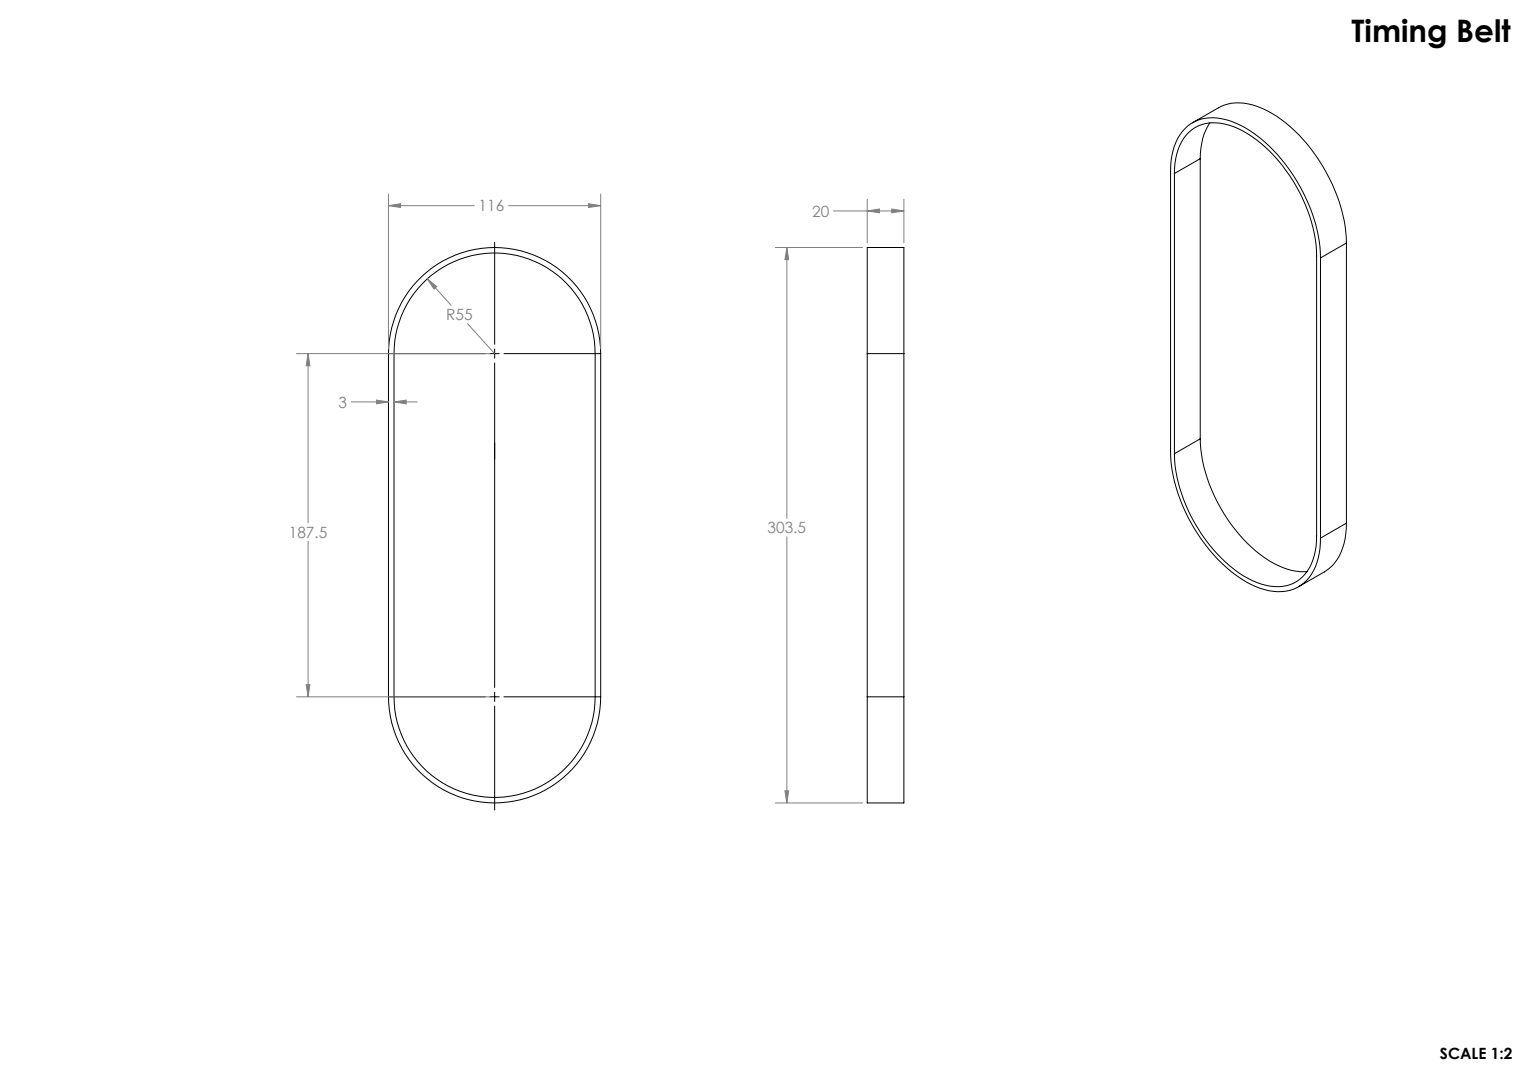
ISO-10303-21;
HEADER;
FILE_DESCRIPTION (('STEP AP214'),
    '1' );
FILE_NAME ('Timing belt.step',
    '2026-10-28T15:55:38',
    ( '' ),
    ( '' ),
    'SwSTEP 2.0',
    'SolidWorks 2025',
    '' );
FILE_SCHEMA (( 'AUTOMOTIVE_DESIGN' ));
ENDSEC;

DATA;
#2=ORIENTED_EDGE ( 'NONE', *, *, #4047, .T. ) ;
#7=VERTEX_POINT ( 'NONE', #7464 ) ;
#32=CARTESIAN_POINT ( 'NONE',  ( 10.00000000000000000, -3.448762466456902719E-14, 93.74999999999998579 ) ) ;
#41=DIRECTION ( 'NONE',  ( 1.000000000000000000, 0.000000000000000000, 0.000000000000000000 ) ) ;
#76=EDGE_CURVE ( 'NONE', #6243, #2665, #5580, .T. ) ;
#91=DIRECTION ( 'NONE',  ( 1.000000000000000000, 0.000000000000000000, 0.000000000000000000 ) ) ;
#104=VECTOR ( 'NONE', #547, 1000.000000000000000 ) ;
#178=CARTESIAN_POINT ( 'NONE',  ( -10.00000000000000000, 2.291769404546313661E-14, -93.74999999999998579 ) ) ;
#186=CARTESIAN_POINT ( 'NONE',  ( 10.00000000000000000, 54.99999999999989342, 93.75000000000004263 ) ) ;
#203=LINE ( 'NONE', #4083, #5436 ) ;
#210=VERTEX_POINT ( 'NONE', #4338 ) ;
#211=MECHANICAL_DESIGN_GEOMETRIC_PRESENTATION_REPRESENTATION('',(#3862),#2523);
#237=ORIENTED_EDGE ( 'NONE', *, *, #6341, .T. ) ;
#282=DIRECTION ( 'NONE',  ( -0.000000000000000000, 1.000000000000000000, 2.960594732333750610E-16 ) ) ;
#285=CARTESIAN_POINT ( 'NONE',  ( 10.00000000000000000, -3.448762466456902719E-14, 93.74999999999998579 ) ) ;
#305=CARTESIAN_POINT ( 'NONE',  ( 10.00000000000000000, -57.99999999999995737, -93.75000000000001421 ) ) ;
#337=CARTESIAN_POINT ( 'NONE',  ( 10.00000000000000000, -57.99999999999995737, -93.75000000000001421 ) ) ;
#343=ADVANCED_FACE ( 'NONE', ( #2220 ), #2779, .T. ) ;
#364=AXIS2_PLACEMENT_3D ( 'NONE', #8155, #2383, #3917 ) ;
#374=EDGE_LOOP ( 'NONE', ( #2417, #694, #4640, #1560, #2095 ) ) ;
#375=ORIENTED_EDGE ( 'NONE', *, *, #4047, .F. ) ;
#376=VECTOR ( 'NONE', #1952, 1000.000000000000000 ) ;
#391=VECTOR ( 'NONE', #4376, 1000.000000000000000 ) ;
#404=CYLINDRICAL_SURFACE ( 'NONE', #1048, 54.99999999999995026 ) ;
#425=( LENGTH_UNIT ( ) NAMED_UNIT ( * ) SI_UNIT ( .MILLI., .METRE. ) );
#429=PLANE ( 'NONE',  #5764 ) ;
#447=AXIS2_PLACEMENT_3D ( 'NONE', #5326, #6108, #2222 ) ;
#460=EDGE_CURVE ( 'NONE', #4967, #5007, #866, .T. ) ;
#473=EDGE_LOOP ( 'NONE', ( #7850, #7709, #1051, #6786 ) ) ;
#483=CARTESIAN_POINT ( 'NONE',  ( -10.00000000000000000, 2.291769404546313661E-14, -93.74999999999998579 ) ) ;
#497=CARTESIAN_POINT ( 'NONE',  ( 10.00000000000000000, -3.448762466456902719E-14, 148.7499999999999432 ) ) ;
#547=DIRECTION ( 'NONE',  ( -1.000000000000000000, -0.000000000000000000, -0.000000000000000000 ) ) ;
#636=ORIENTED_EDGE ( 'NONE', *, *, #7056, .T. ) ;
#637=ORIENTED_EDGE ( 'NONE', *, *, #6590, .T. ) ;
#671=CIRCLE ( 'NONE', #3474, 57.99999999999995737 ) ;
#694=ORIENTED_EDGE ( 'NONE', *, *, #5974, .T. ) ;
#713=AXIS2_PLACEMENT_3D ( 'NONE', #6201, #3523, #6104 ) ;
#718=VERTEX_POINT ( 'NONE', #4108 ) ;
#724=DIRECTION ( 'NONE',  ( 0.000000000000000000, 0.000000000000000000, -1.000000000000000000 ) ) ;
#727=CARTESIAN_POINT ( 'NONE',  ( 10.00000000000000000, 57.99999999999990052, 93.75000000000004263 ) ) ;
#743=FACE_OUTER_BOUND ( 'NONE', #5654, .T. ) ;
#769=ADVANCED_FACE ( 'NONE', ( #2765 ), #1004, .T. ) ;
#803=VECTOR ( 'NONE', #819, 1000.000000000000000 ) ;
#819=DIRECTION ( 'NONE',  ( 0.000000000000000000, -2.960594732333750117E-16, 1.000000000000000000 ) ) ;
#830=EDGE_CURVE ( 'NONE', #718, #2876, #7035, .T. ) ;
#855=CARTESIAN_POINT ( 'NONE',  ( -10.00000000000000000, 57.99999999999997868, -93.74999999999997158 ) ) ;
#862=ADVANCED_FACE ( 'NONE', ( #7728 ), #3981, .F. ) ;
#866=CIRCLE ( 'NONE', #4079, 57.99999999999995737 ) ;
#882=DIRECTION ( 'NONE',  ( -1.000000000000000000, -0.000000000000000000, -0.000000000000000000 ) ) ;
#916=CARTESIAN_POINT ( 'NONE',  ( 10.00000000000000000, 54.99999999999989342, 93.75000000000004263 ) ) ;
#940=PLANE ( 'NONE',  #4467 ) ;
#953=AXIS2_PLACEMENT_3D ( 'NONE', #32, #3926, #724 ) ;
#955=DIRECTION ( 'NONE',  ( 0.000000000000000000, 1.000000000000000000, 0.000000000000000000 ) ) ;
#957=DIRECTION ( 'NONE',  ( 0.000000000000000000, 0.000000000000000000, 1.000000000000000000 ) ) ;
#1004=PLANE ( 'NONE',  #6801 ) ;
#1016=PRODUCT_DEFINITION_SHAPE ( 'NONE', 'NONE',  #2224 ) ;
#1019=CARTESIAN_POINT ( 'NONE',  ( 10.00000000000000000, -54.99999999999995026, -93.75000000000001421 ) ) ;
#1031=DIRECTION ( 'NONE',  ( 1.000000000000000000, 0.000000000000000000, 0.000000000000000000 ) ) ;
#1048=AXIS2_PLACEMENT_3D ( 'NONE', #2974, #882, #3013 ) ;
#1049=VERTEX_POINT ( 'NONE', #727 ) ;
#1051=ORIENTED_EDGE ( 'NONE', *, *, #6903, .T. ) ;
#1054=AXIS2_PLACEMENT_3D ( 'NONE', #285, #3489, #6881 ) ;
#1081=EDGE_LOOP ( 'NONE', ( #2, #4195, #4261, #5785 ) ) ;
#1083=ORIENTED_EDGE ( 'NONE', *, *, #5820, .T. ) ;
#1084=DIRECTION ( 'NONE',  ( 1.000000000000000000, 0.000000000000000000, 0.000000000000000000 ) ) ;
#1127=DIRECTION ( 'NONE',  ( 0.000000000000000000, 1.000000000000000000, 0.000000000000000000 ) ) ;
#1129=ORIENTED_EDGE ( 'NONE', *, *, #2836, .T. ) ;
#1181=ORIENTED_EDGE ( 'NONE', *, *, #460, .F. ) ;
#1209=ADVANCED_FACE ( 'NONE', ( #4121 ), #940, .F. ) ;
#1217=AXIS2_PLACEMENT_3D ( 'NONE', #4251, #1031, #955 ) ;
#1248=EDGE_CURVE ( 'NONE', #5610, #6841, #1936, .T. ) ;
#1281=VERTEX_POINT ( 'NONE', #7607 ) ;
#1299=AXIS2_PLACEMENT_3D ( 'NONE', #5884, #1507, #5927 ) ;
#1328=AXIS2_PLACEMENT_3D ( 'NONE', #6203, #8194, #6070 ) ;
#1345=DIRECTION ( 'NONE',  ( 0.000000000000000000, 0.000000000000000000, -1.000000000000000000 ) ) ;
#1354=CIRCLE ( 'NONE', #953, 54.99999999999995026 ) ;
#1359=EDGE_CURVE ( 'NONE', #6841, #7108, #5297, .T. ) ;
#1387=PLANE ( 'NONE',  #8067 ) ;
#1393=ADVANCED_FACE ( 'NONE', ( #3181 ), #7052, .T. ) ;
#1400=ADVANCED_BREP_SHAPE_REPRESENTATION ( '', ( #3727, #1299 ), #2092 ) ;
#1464=EDGE_LOOP ( 'NONE', ( #4892, #7973, #375, #6797, #1181 ) ) ;
#1470=DIRECTION ( 'NONE',  ( -1.000000000000000000, -0.000000000000000000, -0.000000000000000000 ) ) ;
#1507=DIRECTION ( 'NONE',  ( 0.000000000000000000, 0.000000000000000000, 1.000000000000000000 ) ) ;
#1560=ORIENTED_EDGE ( 'NONE', *, *, #3024, .T. ) ;
#1579=CARTESIAN_POINT ( 'NONE',  ( 10.00000000000000000, 54.99999999999989342, 93.75000000000004263 ) ) ;
#1595=DIRECTION ( 'NONE',  ( 0.000000000000000000, 0.000000000000000000, -1.000000000000000000 ) ) ;
#1623=DIRECTION ( 'NONE',  ( -1.000000000000000000, -0.000000000000000000, -0.000000000000000000 ) ) ;
#1632=EDGE_LOOP ( 'NONE', ( #4319, #5593, #637, #1129, #7242 ) ) ;
#1683=SHAPE_DEFINITION_REPRESENTATION ( #1016, #4267 ) ;
#1697=ORIENTED_EDGE ( 'NONE', *, *, #3134, .T. ) ;
#1738=EDGE_LOOP ( 'NONE', ( #3789, #2490, #5915, #3472 ) ) ;
#1743=VECTOR ( 'NONE', #4143, 1000.000000000000000 ) ;
#1760=AXIS2_PLACEMENT_3D ( 'NONE', #4212, #4859, #4093 ) ;
#1821=LINE ( 'NONE', #4366, #7542 ) ;
#1833=LINE ( 'NONE', #6369, #391 ) ;
#1844=DIRECTION ( 'NONE',  ( 0.000000000000000000, 1.000000000000000000, 0.000000000000000000 ) ) ;
#1934=SHAPE_REPRESENTATION_RELATIONSHIP ( 'NONE' , 'NONE' ,  #4267, #1400 ) ;
#1936=CIRCLE ( 'NONE', #713, 54.99999999999995026 ) ;
#1943=DIRECTION ( 'NONE',  ( 0.000000000000000000, -1.000000000000000000, -2.960594732333750117E-16 ) ) ;
#1952=DIRECTION ( 'NONE',  ( 0.000000000000000000, 2.960594732333750610E-16, -1.000000000000000000 ) ) ;
#1977=( NAMED_UNIT ( * ) SI_UNIT ( $, .STERADIAN. ) SOLID_ANGLE_UNIT ( ) );
#1998=LINE ( 'NONE', #7601, #376 ) ;
#2024=ORIENTED_EDGE ( 'NONE', *, *, #4512, .F. ) ;
#2073=DIRECTION ( 'NONE',  ( 0.000000000000000000, 1.000000000000000000, 0.000000000000000000 ) ) ;
#2086=LINE ( 'NONE', #916, #3884 ) ;
#2092=( GEOMETRIC_REPRESENTATION_CONTEXT ( 3 ) GLOBAL_UNCERTAINTY_ASSIGNED_CONTEXT ( ( #4446 ) ) GLOBAL_UNIT_ASSIGNED_CONTEXT ( ( #5803, #7719, #1977 ) ) REPRESENTATION_CONTEXT ( 'NONE', 'WORKASPACE' ) );
#2095=ORIENTED_EDGE ( 'NONE', *, *, #6647, .T. ) ;
#2220=FACE_OUTER_BOUND ( 'NONE', #1081, .T. ) ;
#2222=DIRECTION ( 'NONE',  ( 0.000000000000000000, 0.000000000000000000, -1.000000000000000000 ) ) ;
#2224=PRODUCT_DEFINITION ( 'UNKNOWN', '', #3672, #7341 ) ;
#2272=VECTOR ( 'NONE', #2306, 1000.000000000000000 ) ;
#2306=DIRECTION ( 'NONE',  ( -1.000000000000000000, -0.000000000000000000, -0.000000000000000000 ) ) ;
#2330=DIRECTION ( 'NONE',  ( 0.000000000000000000, 2.960594732333750610E-16, -1.000000000000000000 ) ) ;
#2383=DIRECTION ( 'NONE',  ( 1.000000000000000000, 0.000000000000000000, 0.000000000000000000 ) ) ;
#2385=( NAMED_UNIT ( * ) SI_UNIT ( $, .STERADIAN. ) SOLID_ANGLE_UNIT ( ) );
#2417=ORIENTED_EDGE ( 'NONE', *, *, #7552, .T. ) ;
#2421=DIRECTION ( 'NONE',  ( 0.000000000000000000, 0.000000000000000000, 1.000000000000000000 ) ) ;
#2490=ORIENTED_EDGE ( 'NONE', *, *, #6181, .F. ) ;
#2498=ORIENTED_EDGE ( 'NONE', *, *, #6788, .T. ) ;
#2523=( GEOMETRIC_REPRESENTATION_CONTEXT ( 3 ) GLOBAL_UNCERTAINTY_ASSIGNED_CONTEXT ( ( #8097 ) ) GLOBAL_UNIT_ASSIGNED_CONTEXT ( ( #425, #7400, #2385 ) ) REPRESENTATION_CONTEXT ( 'NONE', 'WORKASPACE' ) );
#2548=ADVANCED_FACE ( 'NONE', ( #6186 ), #404, .F. ) ;
#2569=CARTESIAN_POINT ( 'NONE',  ( 10.00000000000000000, -3.448762466456902719E-14, 93.74999999999998579 ) ) ;
#2608=DIRECTION ( 'NONE',  ( 0.000000000000000000, 2.960594732333750117E-16, -1.000000000000000000 ) ) ;
#2624=ORIENTED_EDGE ( 'NONE', *, *, #4419, .T. ) ;
#2648=DIRECTION ( 'NONE',  ( 1.000000000000000000, 0.000000000000000000, 0.000000000000000000 ) ) ;
#2665=VERTEX_POINT ( 'NONE', #8308 ) ;
#2682=VECTOR ( 'NONE', #2330, 1000.000000000000000 ) ;
#2724=FACE_OUTER_BOUND ( 'NONE', #1464, .T. ) ;
#2765=FACE_OUTER_BOUND ( 'NONE', #5148, .T. ) ;
#2779=CYLINDRICAL_SURFACE ( 'NONE', #3007, 57.99999999999995737 ) ;
#2806=CARTESIAN_POINT ( 'NONE',  ( -10.00000000000000000, 57.99999999999990052, 93.75000000000004263 ) ) ;
#2836=EDGE_CURVE ( 'NONE', #5161, #4485, #6155, .T. ) ;
#2876=VERTEX_POINT ( 'NONE', #305 ) ;
#2968=EDGE_LOOP ( 'NONE', ( #5843, #2498, #7900, #4205 ) ) ;
#2974=CARTESIAN_POINT ( 'NONE',  ( 10.00000000000000000, -3.448762466456902719E-14, 93.74999999999998579 ) ) ;
#2981=CARTESIAN_POINT ( 'NONE',  ( 10.00000000000000000, 57.99999999999990052, 93.75000000000004263 ) ) ;
#2983=ORIENTED_EDGE ( 'NONE', *, *, #6855, .T. ) ;
#2984=PRODUCT_CONTEXT ( 'NONE', #6112, 'mechanical' ) ;
#3007=AXIS2_PLACEMENT_3D ( 'NONE', #5359, #3440, #2421 ) ;
#3011=DIRECTION ( 'NONE',  ( 0.000000000000000000, -2.960594732333750117E-16, 1.000000000000000000 ) ) ;
#3013=DIRECTION ( 'NONE',  ( 0.000000000000000000, 0.000000000000000000, 1.000000000000000000 ) ) ;
#3024=EDGE_CURVE ( 'NONE', #2876, #8288, #7254, .T. ) ;
#3080=LINE ( 'NONE', #5662, #6442 ) ;
#3090=CARTESIAN_POINT ( 'NONE',  ( 10.00000000000000000, 57.99999999999997868, -93.74999999999997158 ) ) ;
#3107=CARTESIAN_POINT ( 'NONE',  ( -10.00000000000000000, -58.00000000000000711, 93.74999999999998579 ) ) ;
#3127=AXIS2_PLACEMENT_3D ( 'NONE', #7811, #2648, #3263 ) ;
#3134=EDGE_CURVE ( 'NONE', #4302, #5610, #2086, .T. ) ;
#3158=AXIS2_PLACEMENT_3D ( 'NONE', #3340, #1943, #2608 ) ;
#3178=LINE ( 'NONE', #3107, #7784 ) ;
#3181=FACE_OUTER_BOUND ( 'NONE', #2968, .T. ) ;
#3183=VERTEX_POINT ( 'NONE', #2806 ) ;
#3229=ORIENTED_EDGE ( 'NONE', *, *, #1359, .F. ) ;
#3263=DIRECTION ( 'NONE',  ( 0.000000000000000000, 0.000000000000000000, -1.000000000000000000 ) ) ;
#3279=EDGE_CURVE ( 'NONE', #2665, #4302, #5472, .T. ) ;
#3297=DIRECTION ( 'NONE',  ( 0.000000000000000000, 0.000000000000000000, 1.000000000000000000 ) ) ;
#3340=CARTESIAN_POINT ( 'NONE',  ( 10.00000000000000000, 57.99999999999990052, 93.75000000000004263 ) ) ;
#3351=CARTESIAN_POINT ( 'NONE',  ( 10.00000000000000000, 57.99999999999990052, 93.75000000000004263 ) ) ;
#3423=ORIENTED_EDGE ( 'NONE', *, *, #7056, .F. ) ;
#3440=DIRECTION ( 'NONE',  ( -1.000000000000000000, -0.000000000000000000, -0.000000000000000000 ) ) ;
#3472=ORIENTED_EDGE ( 'NONE', *, *, #6646, .T. ) ;
#3473=CIRCLE ( 'NONE', #4830, 54.99999999999995026 ) ;
#3474=AXIS2_PLACEMENT_3D ( 'NONE', #5597, #41, #1844 ) ;
#3489=DIRECTION ( 'NONE',  ( -1.000000000000000000, -0.000000000000000000, -0.000000000000000000 ) ) ;
#3497=ADVANCED_FACE ( 'NONE', ( #7412 ), #6852, .F. ) ;
#3523=DIRECTION ( 'NONE',  ( 1.000000000000000000, 0.000000000000000000, 0.000000000000000000 ) ) ;
#3555=DIRECTION ( 'NONE',  ( 0.000000000000000000, -1.000000000000000000, -2.960594732333750117E-16 ) ) ;
#3622=ORIENTED_EDGE ( 'NONE', *, *, #5152, .T. ) ;
#3672=PRODUCT_DEFINITION_FORMATION_WITH_SPECIFIED_SOURCE ( 'ANY', '', #7957, .NOT_KNOWN. ) ;
#3727=MANIFOLD_SOLID_BREP ( 'Extrude-Thin1', #5441 ) ;
#3737=CARTESIAN_POINT ( 'NONE',  ( 10.00000000000000000, 57.99999999999997868, -93.74999999999997158 ) ) ;
#3747=CARTESIAN_POINT ( 'NONE',  ( -10.00000000000000000, -3.448762466456902719E-14, 148.7499999999999432 ) ) ;
#3789=ORIENTED_EDGE ( 'NONE', *, *, #6590, .F. ) ;
#3829=ORIENTED_EDGE ( 'NONE', *, *, #1248, .F. ) ;
#3862=STYLED_ITEM('',(#8407),#3727);
#3866=EDGE_LOOP ( 'NONE', ( #5583, #6325, #7669, #2624 ) ) ;
#3884=VECTOR ( 'NONE', #1470, 1000.000000000000000 ) ;
#3917=DIRECTION ( 'NONE',  ( 0.000000000000000000, 1.000000000000000000, 0.000000000000000000 ) ) ;
#3926=DIRECTION ( 'NONE',  ( 1.000000000000000000, 0.000000000000000000, 0.000000000000000000 ) ) ;
#3958=ORIENTED_EDGE ( 'NONE', *, *, #6646, .F. ) ;
#3981=PLANE ( 'NONE',  #3158 ) ;
#4014=VECTOR ( 'NONE', #6749, 1000.000000000000000 ) ;
#4025=FACE_BOUND ( 'NONE', #1632, .T. ) ;
#4042=CARTESIAN_POINT ( 'NONE',  ( -10.00000000000000000, 57.99999999999990052, 93.75000000000004263 ) ) ;
#4047=EDGE_CURVE ( 'NONE', #210, #8056, #6564, .T. ) ;
#4079=AXIS2_PLACEMENT_3D ( 'NONE', #5210, #91, #2073 ) ;
#4083=CARTESIAN_POINT ( 'NONE',  ( 10.00000000000000000, -55.00000000000000711, 93.74999999999998579 ) ) ;
#4093=DIRECTION ( 'NONE',  ( 0.000000000000000000, 1.000000000000000000, 0.000000000000000000 ) ) ;
#4108=CARTESIAN_POINT ( 'NONE',  ( 10.00000000000000000, -58.00000000000000711, 93.74999999999998579 ) ) ;
#4121=FACE_OUTER_BOUND ( 'NONE', #7722, .T. ) ;
#4136=DIRECTION ( 'NONE',  ( -1.000000000000000000, -0.000000000000000000, -0.000000000000000000 ) ) ;
#4141=VECTOR ( 'NONE', #4586, 1000.000000000000000 ) ;
#4143=DIRECTION ( 'NONE',  ( -1.000000000000000000, -0.000000000000000000, -0.000000000000000000 ) ) ;
#4165=FACE_OUTER_BOUND ( 'NONE', #473, .T. ) ;
#4183=DIRECTION ( 'NONE',  ( 1.000000000000000000, 0.000000000000000000, 0.000000000000000000 ) ) ;
#4195=ORIENTED_EDGE ( 'NONE', *, *, #4419, .F. ) ;
#4205=ORIENTED_EDGE ( 'NONE', *, *, #6855, .F. ) ;
#4212=CARTESIAN_POINT ( 'NONE',  ( 10.00000000000000000, -3.448762466456902719E-14, 93.74999999999998579 ) ) ;
#4251=CARTESIAN_POINT ( 'NONE',  ( -10.00000000000000000, -3.448762466456902719E-14, 93.74999999999998579 ) ) ;
#4255=ORIENTED_EDGE ( 'NONE', *, *, #76, .T. ) ;
#4261=ORIENTED_EDGE ( 'NONE', *, *, #3024, .F. ) ;
#4262=CARTESIAN_POINT ( 'NONE',  ( -10.00000000000000000, -55.00000000000000711, 93.74999999999998579 ) ) ;
#4267=SHAPE_REPRESENTATION ( 'Timing belt', ( #1299 ), #2092 ) ;
#4302=VERTEX_POINT ( 'NONE', #1579 ) ;
#4319=ORIENTED_EDGE ( 'NONE', *, *, #1248, .T. ) ;
#4338=CARTESIAN_POINT ( 'NONE',  ( -10.00000000000000000, -57.99999999999995737, -93.75000000000001421 ) ) ;
#4339=LINE ( 'NONE', #3090, #2272 ) ;
#4366=CARTESIAN_POINT ( 'NONE',  ( 10.00000000000000000, -3.448762466456902719E-14, 151.7499999999999432 ) ) ;
#4376=DIRECTION ( 'NONE',  ( 0.000000000000000000, -2.960594732333750117E-16, 1.000000000000000000 ) ) ;
#4388=AXIS2_PLACEMENT_3D ( 'NONE', #483, #1084, #1127 ) ;
#4419=EDGE_CURVE ( 'NONE', #8288, #8056, #4339, .T. ) ;
#4446=UNCERTAINTY_MEASURE_WITH_UNIT (LENGTH_MEASURE( 1.000000000000000082E-05 ), #5803, 'distance_accuracy_value', 'NONE');
#4460=ADVANCED_FACE ( 'NONE', ( #6163 ), #429, .T. ) ;
#4467=AXIS2_PLACEMENT_3D ( 'NONE', #6068, #282, #5445 ) ;
#4485=VERTEX_POINT ( 'NONE', #5588 ) ;
#4488=CARTESIAN_POINT ( 'NONE',  ( -10.00000000000000000, 54.99999999999989342, 93.75000000000004263 ) ) ;
#4498=ORIENTED_EDGE ( 'NONE', *, *, #8299, .T. ) ;
#4512=EDGE_CURVE ( 'NONE', #2876, #210, #7406, .T. ) ;
#4526=DIRECTION ( 'NONE',  ( 0.000000000000000000, 0.000000000000000000, 1.000000000000000000 ) ) ;
#4544=VECTOR ( 'NONE', #3011, 1000.000000000000000 ) ;
#4586=DIRECTION ( 'NONE',  ( -1.000000000000000000, -0.000000000000000000, -0.000000000000000000 ) ) ;
#4616=DIRECTION ( 'NONE',  ( 0.000000000000000000, 2.960594732333750610E-16, -1.000000000000000000 ) ) ;
#4625=DIRECTION ( 'NONE',  ( 1.000000000000000000, 0.000000000000000000, 0.000000000000000000 ) ) ;
#4640=ORIENTED_EDGE ( 'NONE', *, *, #830, .T. ) ;
#4744=AXIS2_PLACEMENT_3D ( 'NONE', #2569, #7160, #4526 ) ;
#4781=CARTESIAN_POINT ( 'NONE',  ( 10.00000000000000000, 54.99999999999997158, -93.74999999999998579 ) ) ;
#4794=LINE ( 'NONE', #2981, #5101 ) ;
#4830=AXIS2_PLACEMENT_3D ( 'NONE', #7377, #4183, #1595 ) ;
#4838=CIRCLE ( 'NONE', #1217, 57.99999999999995737 ) ;
#4859=DIRECTION ( 'NONE',  ( 1.000000000000000000, 0.000000000000000000, 0.000000000000000000 ) ) ;
#4886=ADVANCED_FACE ( 'NONE', ( #4165 ), #8107, .T. ) ;
#4892=ORIENTED_EDGE ( 'NONE', *, *, #7590, .F. ) ;
#4920=ORIENTED_EDGE ( 'NONE', *, *, #5820, .F. ) ;
#4936=ADVANCED_FACE ( 'NONE', ( #6151, #4976 ), #6838, .T. ) ;
#4967=VERTEX_POINT ( 'NONE', #8059 ) ;
#4976=FACE_BOUND ( 'NONE', #5251, .T. ) ;
#5007=VERTEX_POINT ( 'NONE', #7011 ) ;
#5101=VECTOR ( 'NONE', #7388, 1000.000000000000000 ) ;
#5127=DIRECTION ( 'NONE',  ( 0.000000000000000000, 2.960594732333750610E-16, -1.000000000000000000 ) ) ;
#5138=DIRECTION ( 'NONE',  ( -1.000000000000000000, -0.000000000000000000, -0.000000000000000000 ) ) ;
#5148=EDGE_LOOP ( 'NONE', ( #6039, #4920, #7842, #1697 ) ) ;
#5152=EDGE_CURVE ( 'NONE', #6778, #6841, #3080, .T. ) ;
#5161=VERTEX_POINT ( 'NONE', #5865 ) ;
#5210=CARTESIAN_POINT ( 'NONE',  ( -10.00000000000000000, -3.448762466456902719E-14, 93.74999999999998579 ) ) ;
#5251=EDGE_LOOP ( 'NONE', ( #7010, #3423, #6746, #6280, #5573 ) ) ;
#5297=CIRCLE ( 'NONE', #3127, 54.99999999999995026 ) ;
#5299=CARTESIAN_POINT ( 'NONE',  ( 10.00000000000000000, -3.448762466456902719E-14, 93.74999999999998579 ) ) ;
#5307=CARTESIAN_POINT ( 'NONE',  ( -10.00000000000000000, -3.448762466456902719E-14, 93.74999999999998579 ) ) ;
#5326=CARTESIAN_POINT ( 'NONE',  ( 10.00000000000000000, 2.291769404546313661E-14, -93.74999999999998579 ) ) ;
#5359=CARTESIAN_POINT ( 'NONE',  ( 10.00000000000000000, 2.291769404546313661E-14, -93.74999999999998579 ) ) ;
#5422=DIRECTION ( 'NONE',  ( 1.000000000000000000, 0.000000000000000000, 0.000000000000000000 ) ) ;
#5436=VECTOR ( 'NONE', #7984, 1000.000000000000000 ) ;
#5441=CLOSED_SHELL ( 'NONE', ( #2548, #1393, #4936, #5672, #4886, #1209, #343, #862, #7373, #4460, #3497, #769 ) ) ;
#5445=DIRECTION ( 'NONE',  ( 0.000000000000000000, -2.960594732333750610E-16, 1.000000000000000000 ) ) ;
#5450=LINE ( 'NONE', #4042, #803 ) ;
#5472=LINE ( 'NONE', #6092, #4544 ) ;
#5500=AXIS2_PLACEMENT_3D ( 'NONE', #5548, #4136, #957 ) ;
#5548=CARTESIAN_POINT ( 'NONE',  ( 10.00000000000000000, 2.291769404546313661E-14, -93.74999999999998579 ) ) ;
#5573=ORIENTED_EDGE ( 'NONE', *, *, #76, .F. ) ;
#5580=CIRCLE ( 'NONE', #447, 54.99999999999995026 ) ;
#5583=ORIENTED_EDGE ( 'NONE', *, *, #6113, .T. ) ;
#5588=CARTESIAN_POINT ( 'NONE',  ( -10.00000000000000000, 54.99999999999997158, -93.74999999999998579 ) ) ;
#5590=VECTOR ( 'NONE', #4616, 1000.000000000000000 ) ;
#5593=ORIENTED_EDGE ( 'NONE', *, *, #1359, .T. ) ;
#5597=CARTESIAN_POINT ( 'NONE',  ( 10.00000000000000000, -3.448762466456902719E-14, 93.74999999999998579 ) ) ;
#5608=LINE ( 'NONE', #8186, #4014 ) ;
#5610=VERTEX_POINT ( 'NONE', #4488 ) ;
#5654=EDGE_LOOP ( 'NONE', ( #8150, #636, #6202, #3229 ) ) ;
#5662=CARTESIAN_POINT ( 'NONE',  ( 10.00000000000000000, -3.448762466456902719E-14, 148.7499999999999432 ) ) ;
#5672=ADVANCED_FACE ( 'NONE', ( #2724, #4025 ), #1387, .F. ) ;
#5764=AXIS2_PLACEMENT_3D ( 'NONE', #7532, #6805, #8072 ) ;
#5785=ORIENTED_EDGE ( 'NONE', *, *, #4512, .T. ) ;
#5803=( LENGTH_UNIT ( ) NAMED_UNIT ( * ) SI_UNIT ( .MILLI., .METRE. ) );
#5820=EDGE_CURVE ( 'NONE', #2665, #4485, #6814, .T. ) ;
#5843=ORIENTED_EDGE ( 'NONE', *, *, #5974, .F. ) ;
#5865=CARTESIAN_POINT ( 'NONE',  ( -10.00000000000000000, -54.99999999999995026, -93.75000000000001421 ) ) ;
#5884=CARTESIAN_POINT ( 'NONE',  ( 0.000000000000000000, 0.000000000000000000, 0.000000000000000000 ) ) ;
#5915=ORIENTED_EDGE ( 'NONE', *, *, #6709, .T. ) ;
#5927=DIRECTION ( 'NONE',  ( 1.000000000000000000, 0.000000000000000000, 0.000000000000000000 ) ) ;
#5974=EDGE_CURVE ( 'NONE', #1281, #718, #671, .T. ) ;
#6039=ORIENTED_EDGE ( 'NONE', *, *, #6422, .F. ) ;
#6048=DIRECTION ( 'NONE',  ( 0.000000000000000000, 0.000000000000000000, -1.000000000000000000 ) ) ;
#6068=CARTESIAN_POINT ( 'NONE',  ( 10.00000000000000000, -58.00000000000000711, 93.74999999999998579 ) ) ;
#6070=DIRECTION ( 'NONE',  ( 0.000000000000000000, 0.000000000000000000, -1.000000000000000000 ) ) ;
#6092=CARTESIAN_POINT ( 'NONE',  ( 10.00000000000000000, 54.99999999999989342, 93.75000000000004263 ) ) ;
#6104=DIRECTION ( 'NONE',  ( 0.000000000000000000, 0.000000000000000000, -1.000000000000000000 ) ) ;
#6108=DIRECTION ( 'NONE',  ( 1.000000000000000000, 0.000000000000000000, 0.000000000000000000 ) ) ;
#6112=APPLICATION_CONTEXT ( 'automotive_design' ) ;
#6113=EDGE_CURVE ( 'NONE', #8056, #3183, #5450, .T. ) ;
#6151=FACE_OUTER_BOUND ( 'NONE', #374, .T. ) ;
#6155=CIRCLE ( 'NONE', #7523, 54.99999999999995026 ) ;
#6163=FACE_OUTER_BOUND ( 'NONE', #1738, .T. ) ;
#6181=EDGE_CURVE ( 'NONE', #7, #7108, #203, .T. ) ;
#6186=FACE_OUTER_BOUND ( 'NONE', #7204, .T. ) ;
#6201=CARTESIAN_POINT ( 'NONE',  ( -10.00000000000000000, -3.448762466456902719E-14, 93.74999999999998579 ) ) ;
#6202=ORIENTED_EDGE ( 'NONE', *, *, #6181, .T. ) ;
#6203=CARTESIAN_POINT ( 'NONE',  ( 10.00000000000000000, -3.448762466456902719E-14, 93.74999999999998579 ) ) ;
#6243=VERTEX_POINT ( 'NONE', #1019 ) ;
#6280=ORIENTED_EDGE ( 'NONE', *, *, #3279, .F. ) ;
#6325=ORIENTED_EDGE ( 'NONE', *, *, #6903, .F. ) ;
#6326=CARTESIAN_POINT ( 'NONE',  ( 10.00000000000000000, -58.00000000000000711, 93.74999999999998579 ) ) ;
#6341=EDGE_CURVE ( 'NONE', #4302, #6778, #1354, .T. ) ;
#6369=CARTESIAN_POINT ( 'NONE',  ( -10.00000000000000000, 54.99999999999989342, 93.75000000000004263 ) ) ;
#6398=LINE ( 'NONE', #6326, #104 ) ;
#6422=EDGE_CURVE ( 'NONE', #4485, #5610, #1833, .T. ) ;
#6442=VECTOR ( 'NONE', #7173, 1000.000000000000000 ) ;
#6461=AXIS2_PLACEMENT_3D ( 'NONE', #5299, #7882, #3297 ) ;
#6520=CARTESIAN_POINT ( 'NONE',  ( 10.00000000000000000, -58.00000000000000711, 93.74999999999998579 ) ) ;
#6561=APPLICATION_CONTEXT ( 'automotive_design' ) ;
#6562=CYLINDRICAL_SURFACE ( 'NONE', #6461, 54.99999999999995026 ) ;
#6564=CIRCLE ( 'NONE', #4388, 57.99999999999995737 ) ;
#6590=EDGE_CURVE ( 'NONE', #7108, #5161, #8101, .T. ) ;
#6646=EDGE_CURVE ( 'NONE', #6243, #5161, #5608, .T. ) ;
#6647=EDGE_CURVE ( 'NONE', #8288, #1049, #4794, .T. ) ;
#6709=EDGE_CURVE ( 'NONE', #7, #6243, #1998, .T. ) ;
#6746=ORIENTED_EDGE ( 'NONE', *, *, #6341, .F. ) ;
#6749=DIRECTION ( 'NONE',  ( -1.000000000000000000, -0.000000000000000000, -0.000000000000000000 ) ) ;
#6778=VERTEX_POINT ( 'NONE', #497 ) ;
#6786=ORIENTED_EDGE ( 'NONE', *, *, #7590, .T. ) ;
#6788=EDGE_CURVE ( 'NONE', #1281, #4967, #1821, .T. ) ;
#6797=ORIENTED_EDGE ( 'NONE', *, *, #8299, .F. ) ;
#6801=AXIS2_PLACEMENT_3D ( 'NONE', #186, #3555, #7970 ) ;
#6805=DIRECTION ( 'NONE',  ( -0.000000000000000000, 1.000000000000000000, 2.960594732333750610E-16 ) ) ;
#6814=LINE ( 'NONE', #4781, #1743 ) ;
#6827=CARTESIAN_POINT ( 'NONE',  ( -10.00000000000000000, -55.00000000000000711, 93.74999999999998579 ) ) ;
#6838=PLANE ( 'NONE',  #1328 ) ;
#6841=VERTEX_POINT ( 'NONE', #3747 ) ;
#6852=CYLINDRICAL_SURFACE ( 'NONE', #5500, 54.99999999999995026 ) ;
#6855=EDGE_CURVE ( 'NONE', #718, #5007, #6398, .T. ) ;
#6869=CIRCLE ( 'NONE', #1760, 57.99999999999995737 ) ;
#6881=DIRECTION ( 'NONE',  ( 0.000000000000000000, 0.000000000000000000, 1.000000000000000000 ) ) ;
#6903=EDGE_CURVE ( 'NONE', #1049, #3183, #7207, .T. ) ;
#6976=ORIENTED_EDGE ( 'NONE', *, *, #830, .F. ) ;
#6994=ORIENTED_EDGE ( 'NONE', *, *, #2836, .F. ) ;
#7010=ORIENTED_EDGE ( 'NONE', *, *, #6709, .F. ) ;
#7011=CARTESIAN_POINT ( 'NONE',  ( -10.00000000000000000, -58.00000000000000711, 93.74999999999998579 ) ) ;
#7035=LINE ( 'NONE', #6520, #5590 ) ;
#7052=CYLINDRICAL_SURFACE ( 'NONE', #4744, 57.99999999999995737 ) ;
#7056=EDGE_CURVE ( 'NONE', #6778, #7, #3473, .T. ) ;
#7108=VERTEX_POINT ( 'NONE', #4262 ) ;
#7160=DIRECTION ( 'NONE',  ( -1.000000000000000000, -0.000000000000000000, -0.000000000000000000 ) ) ;
#7173=DIRECTION ( 'NONE',  ( -1.000000000000000000, -0.000000000000000000, -0.000000000000000000 ) ) ;
#7204=EDGE_LOOP ( 'NONE', ( #237, #3622, #3829, #8309 ) ) ;
#7207=LINE ( 'NONE', #3351, #4141 ) ;
#7242=ORIENTED_EDGE ( 'NONE', *, *, #6422, .T. ) ;
#7254=CIRCLE ( 'NONE', #364, 57.99999999999995737 ) ;
#7341=PRODUCT_DEFINITION_CONTEXT ( 'detailed design', #6561, 'design' ) ;
#7373=ADVANCED_FACE ( 'NONE', ( #743 ), #6562, .F. ) ;
#7377=CARTESIAN_POINT ( 'NONE',  ( 10.00000000000000000, -3.448762466456902719E-14, 93.74999999999998579 ) ) ;
#7388=DIRECTION ( 'NONE',  ( 0.000000000000000000, -2.960594732333750117E-16, 1.000000000000000000 ) ) ;
#7400=( NAMED_UNIT ( * ) PLANE_ANGLE_UNIT ( ) SI_UNIT ( $, .RADIAN. ) );
#7406=LINE ( 'NONE', #337, #7518 ) ;
#7412=FACE_OUTER_BOUND ( 'NONE', #8234, .T. ) ;
#7464=CARTESIAN_POINT ( 'NONE',  ( 10.00000000000000000, -55.00000000000000711, 93.74999999999998579 ) ) ;
#7518=VECTOR ( 'NONE', #1623, 1000.000000000000000 ) ;
#7523=AXIS2_PLACEMENT_3D ( 'NONE', #178, #5422, #6048 ) ;
#7532=CARTESIAN_POINT ( 'NONE',  ( 10.00000000000000000, -55.00000000000000711, 93.74999999999998579 ) ) ;
#7542=VECTOR ( 'NONE', #5138, 1000.000000000000000 ) ;
#7552=EDGE_CURVE ( 'NONE', #1049, #1281, #6869, .T. ) ;
#7590=EDGE_CURVE ( 'NONE', #3183, #4967, #4838, .T. ) ;
#7601=CARTESIAN_POINT ( 'NONE',  ( 10.00000000000000000, -55.00000000000000711, 93.74999999999998579 ) ) ;
#7607=CARTESIAN_POINT ( 'NONE',  ( 10.00000000000000000, -3.448762466456902719E-14, 151.7499999999999432 ) ) ;
#7669=ORIENTED_EDGE ( 'NONE', *, *, #6647, .F. ) ;
#7709=ORIENTED_EDGE ( 'NONE', *, *, #7552, .F. ) ;
#7719=( NAMED_UNIT ( * ) PLANE_ANGLE_UNIT ( ) SI_UNIT ( $, .RADIAN. ) );
#7722=EDGE_LOOP ( 'NONE', ( #4498, #2024, #6976, #2983 ) ) ;
#7728=FACE_OUTER_BOUND ( 'NONE', #3866, .T. ) ;
#7784=VECTOR ( 'NONE', #5127, 1000.000000000000000 ) ;
#7811=CARTESIAN_POINT ( 'NONE',  ( -10.00000000000000000, -3.448762466456902719E-14, 93.74999999999998579 ) ) ;
#7842=ORIENTED_EDGE ( 'NONE', *, *, #3279, .T. ) ;
#7850=ORIENTED_EDGE ( 'NONE', *, *, #6788, .F. ) ;
#7882=DIRECTION ( 'NONE',  ( -1.000000000000000000, -0.000000000000000000, -0.000000000000000000 ) ) ;
#7900=ORIENTED_EDGE ( 'NONE', *, *, #460, .T. ) ;
#7957=PRODUCT ( 'Timing belt', 'Timing belt', '', ( #2984 ) ) ;
#7970=DIRECTION ( 'NONE',  ( 0.000000000000000000, 2.960594732333750117E-16, -1.000000000000000000 ) ) ;
#7973=ORIENTED_EDGE ( 'NONE', *, *, #6113, .F. ) ;
#7984=DIRECTION ( 'NONE',  ( -1.000000000000000000, -0.000000000000000000, -0.000000000000000000 ) ) ;
#8056=VERTEX_POINT ( 'NONE', #855 ) ;
#8059=CARTESIAN_POINT ( 'NONE',  ( -10.00000000000000000, -3.448762466456902719E-14, 151.7499999999999432 ) ) ;
#8067=AXIS2_PLACEMENT_3D ( 'NONE', #5307, #4625, #1345 ) ;
#8072=DIRECTION ( 'NONE',  ( 0.000000000000000000, -2.960594732333750610E-16, 1.000000000000000000 ) ) ;
#8097=UNCERTAINTY_MEASURE_WITH_UNIT (LENGTH_MEASURE( 1.000000000000000082E-05 ), #425, 'distance_accuracy_value', 'NONE');
#8101=LINE ( 'NONE', #6827, #2682 ) ;
#8107=CYLINDRICAL_SURFACE ( 'NONE', #1054, 57.99999999999995737 ) ;
#8150=ORIENTED_EDGE ( 'NONE', *, *, #5152, .F. ) ;
#8155=CARTESIAN_POINT ( 'NONE',  ( 10.00000000000000000, 2.291769404546313661E-14, -93.74999999999998579 ) ) ;
#8186=CARTESIAN_POINT ( 'NONE',  ( 10.00000000000000000, -54.99999999999995026, -93.75000000000001421 ) ) ;
#8194=DIRECTION ( 'NONE',  ( 1.000000000000000000, 0.000000000000000000, 0.000000000000000000 ) ) ;
#8234=EDGE_LOOP ( 'NONE', ( #6994, #3958, #4255, #1083 ) ) ;
#8288=VERTEX_POINT ( 'NONE', #3737 ) ;
#8299=EDGE_CURVE ( 'NONE', #5007, #210, #3178, .T. ) ;
#8308=CARTESIAN_POINT ( 'NONE',  ( 10.00000000000000000, 54.99999999999995026, -93.74999999999997158 ) ) ;
#8309=ORIENTED_EDGE ( 'NONE', *, *, #3134, .F. ) ;
#8401=COLOUR_RGB('Black',0.12,0.14,0.17);
#8402=FILL_AREA_STYLE_COLOUR('',#8401);
#8403=FILL_AREA_STYLE('',(#8402));
#8404=SURFACE_STYLE_FILL_AREA(#8403);
#8405=SURFACE_SIDE_STYLE('',(#8404));
#8406=SURFACE_STYLE_USAGE(.BOTH.,#8405);
#8407=PRESENTATION_STYLE_ASSIGNMENT((#8406));
ENDSEC;
END-ISO-10303-21;
